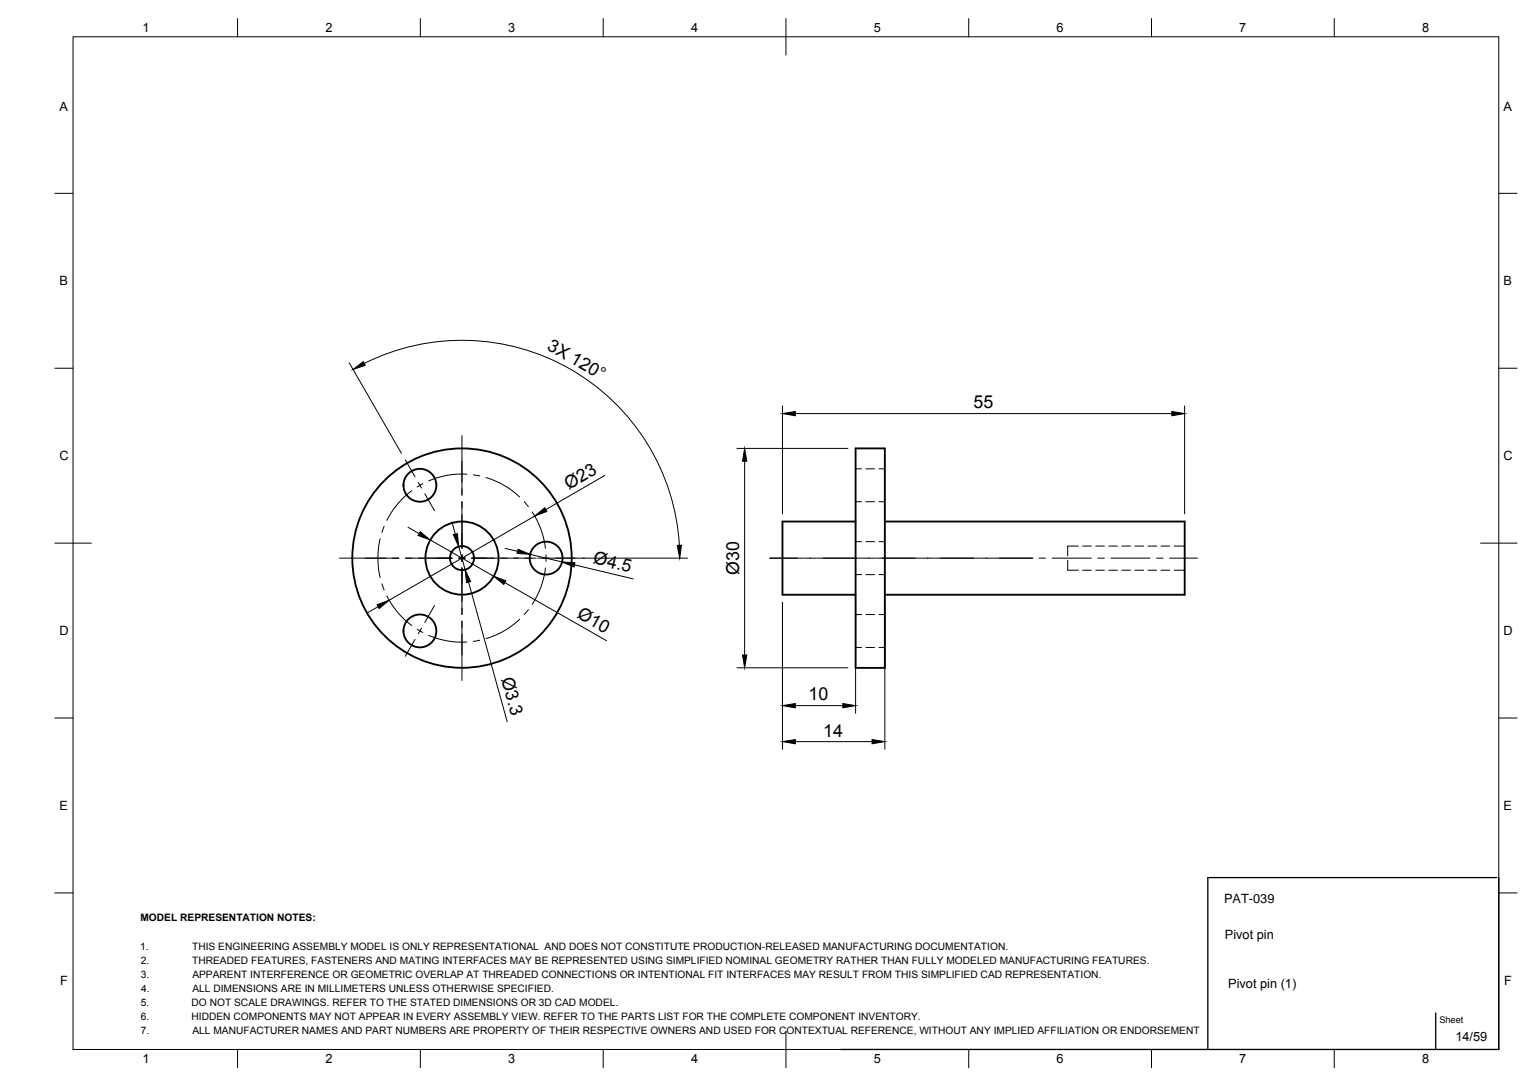
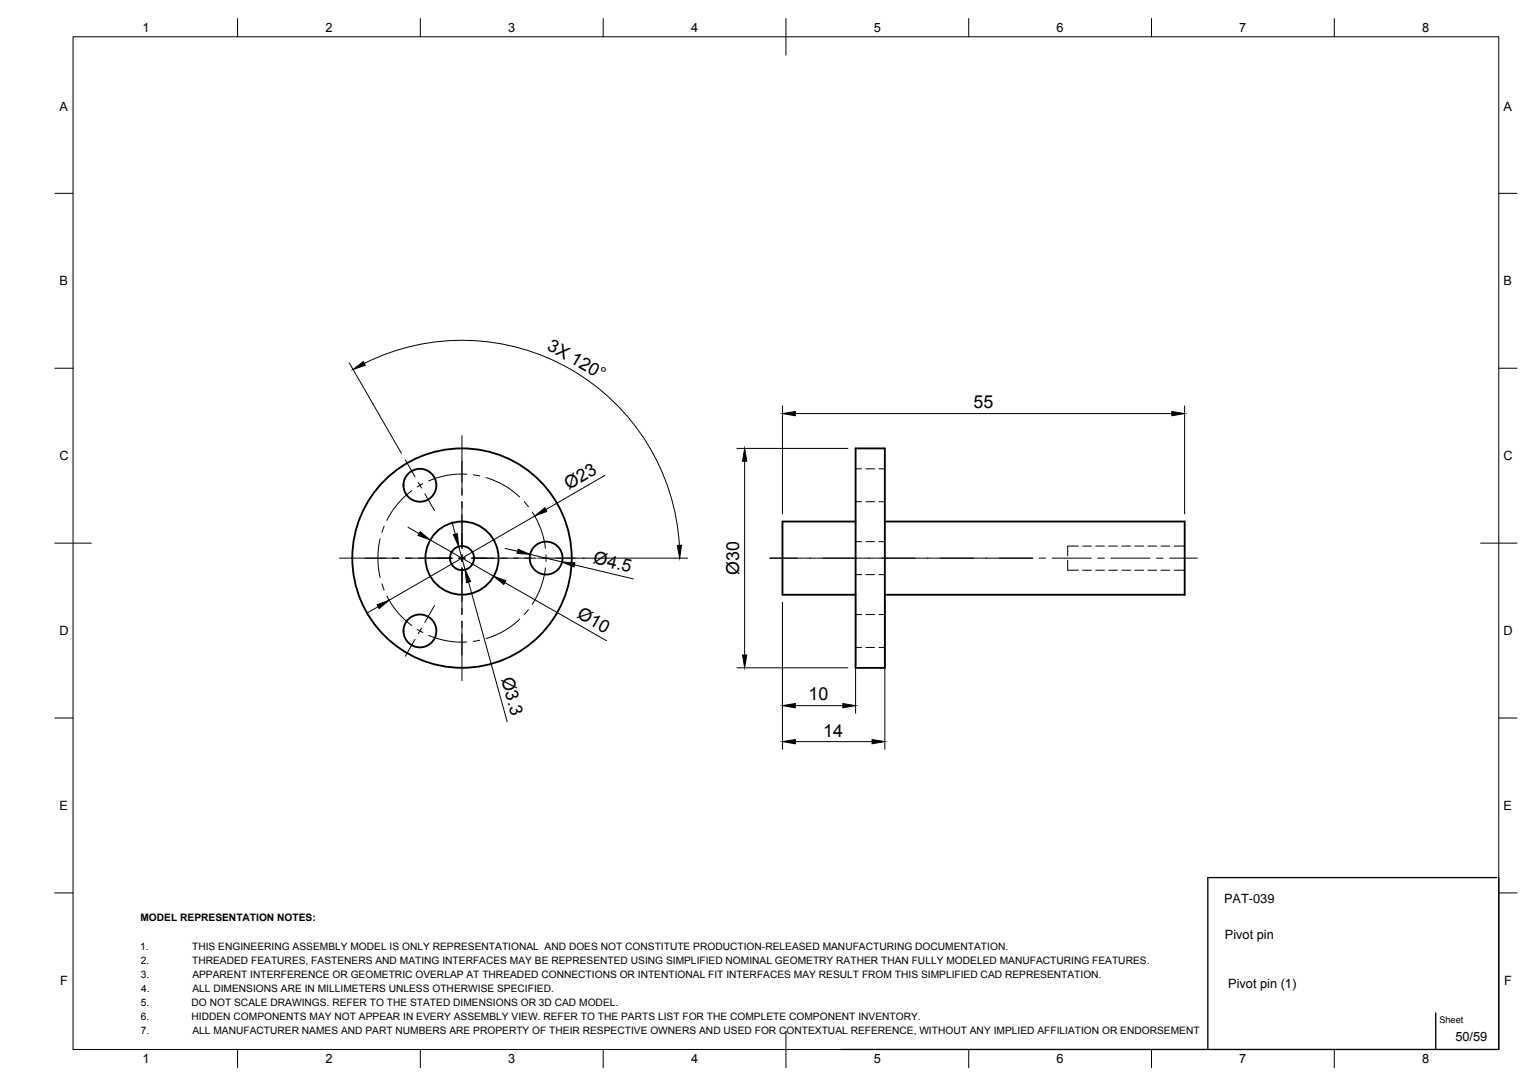
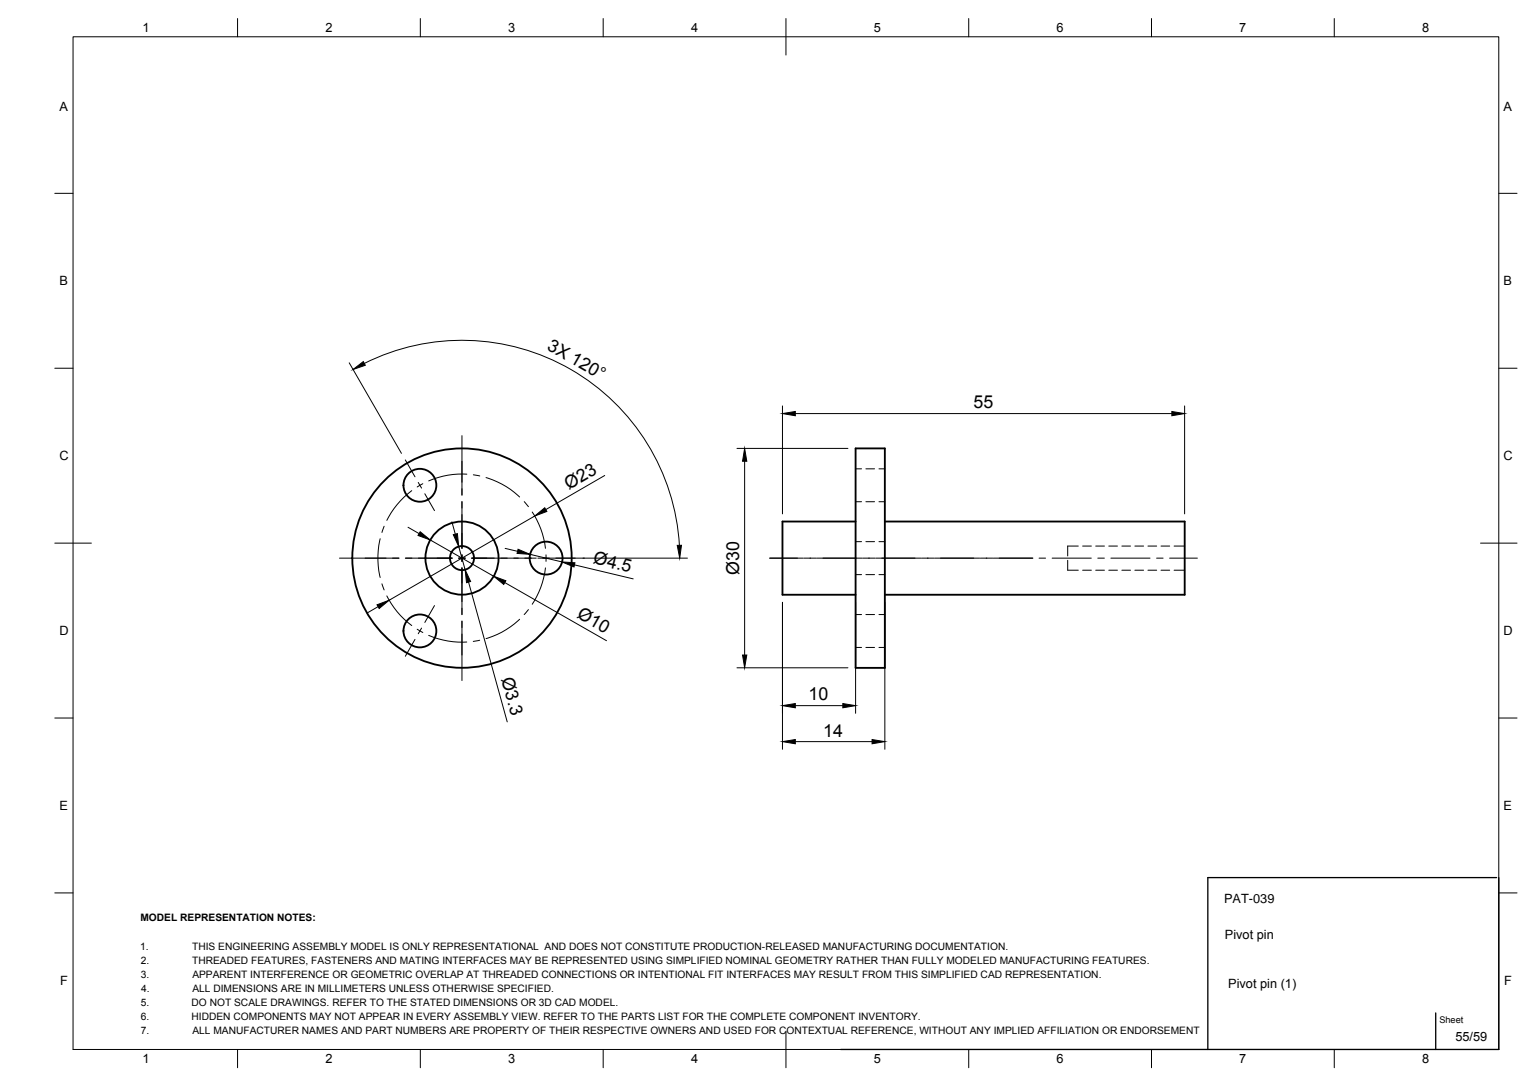
ISO-10303-21;
HEADER;
/* Generated by software containing ST-Developer
 * from STEP Tools, Inc. (www.steptools.com) 
 */

FILE_DESCRIPTION(
/* description */ ('Four-bar parallelogram arm'),
/* implementation_level */ '2;1');

FILE_NAME(
/* name */ 'Pivot pin.step',
/* time_stamp */ '2026-10-28T03:24:55-07:00',
/* author */ (''),
/* organization */ (''),
/* preprocessor_version */ 'ST-DEVELOPER v20.2',
/* originating_system */ 'Autodesk Translation Framework v15.17.0.0',
/* authorisation */ '');

FILE_SCHEMA (('AUTOMOTIVE_DESIGN { 1 0 10303 214 3 1 1 }'));
ENDSEC;

DATA;
#10=MECHANICAL_DESIGN_GEOMETRIC_PRESENTATION_REPRESENTATION('',(#631),#14512);
#531=SHAPE_REPRESENTATION_RELATIONSHIP('SRR','None',#14752,#581);
#581=ADVANCED_BREP_SHAPE_REPRESENTATION('',(#689),#14467);
#631=STYLED_ITEM('',(#15087),#689);
#689=MANIFOLD_SOLID_BREP('Body1',#7335);
#785=FACE_BOUND('',#1751,.T.);
#786=FACE_BOUND('',#1752,.T.);
#787=FACE_BOUND('',#1753,.T.);
#788=FACE_BOUND('',#1754,.T.);
#789=FACE_BOUND('',#1756,.T.);
#790=FACE_BOUND('',#1757,.T.);
#791=FACE_BOUND('',#1758,.T.);
#792=FACE_BOUND('',#1759,.T.);
#793=FACE_BOUND('',#1765,.T.);
#1048=PLANE('',#8091);
#1049=PLANE('',#8101);
#1050=PLANE('',#8104);
#1051=PLANE('',#8112);
#1052=PLANE('',#8113);
#1275=FACE_OUTER_BOUND('',#1745,.T.);
#1276=FACE_OUTER_BOUND('',#1746,.T.);
#1277=FACE_OUTER_BOUND('',#1747,.T.);
#1278=FACE_OUTER_BOUND('',#1748,.T.);
#1279=FACE_OUTER_BOUND('',#1749,.T.);
#1280=FACE_OUTER_BOUND('',#1750,.T.);
#1281=FACE_OUTER_BOUND('',#1755,.T.);
#1282=FACE_OUTER_BOUND('',#1760,.T.);
#1283=FACE_OUTER_BOUND('',#1761,.T.);
#1284=FACE_OUTER_BOUND('',#1762,.T.);
#1285=FACE_OUTER_BOUND('',#1763,.T.);
#1286=FACE_OUTER_BOUND('',#1764,.T.);
#1745=EDGE_LOOP('',(#5300,#5301,#5302,#5303));
#1746=EDGE_LOOP('',(#5304));
#1747=EDGE_LOOP('',(#5305,#5306,#5307,#5308));
#1748=EDGE_LOOP('',(#5309,#5310,#5311,#5312));
#1749=EDGE_LOOP('',(#5313,#5314,#5315,#5316));
#1750=EDGE_LOOP('',(#5317));
#1751=EDGE_LOOP('',(#5318));
#1752=EDGE_LOOP('',(#5319));
#1753=EDGE_LOOP('',(#5320));
#1754=EDGE_LOOP('',(#5321));
#1755=EDGE_LOOP('',(#5322));
#1756=EDGE_LOOP('',(#5323));
#1757=EDGE_LOOP('',(#5324));
#1758=EDGE_LOOP('',(#5325));
#1759=EDGE_LOOP('',(#5326));
#1760=EDGE_LOOP('',(#5327,#5328,#5329,#5330));
#1761=EDGE_LOOP('',(#5331,#5332,#5333,#5334));
#1762=EDGE_LOOP('',(#5335,#5336,#5337,#5338));
#1763=EDGE_LOOP('',(#5339));
#1764=EDGE_LOOP('',(#5340));
#1765=EDGE_LOOP('',(#5341));
#2404=LINE('',#11778,#2798);
#2405=LINE('',#11785,#2799);
#2406=LINE('',#11791,#2800);
#2407=LINE('',#11797,#2801);
#2408=LINE('',#11810,#2802);
#2409=LINE('',#11813,#2803);
#2410=LINE('',#11818,#2804);
#2798=VECTOR('',#9366,0.165);
#2799=VECTOR('',#9375,0.225);
#2800=VECTOR('',#9382,0.225);
#2801=VECTOR('',#9389,0.225);
#2802=VECTOR('',#9406,1.5);
#2803=VECTOR('',#9409,0.5);
#2804=VECTOR('',#9416,0.5);
#3164=CIRCLE('',#8089,0.165);
#3165=CIRCLE('',#8090,0.165);
#3166=CIRCLE('',#8093,0.225);
#3167=CIRCLE('',#8094,0.225);
#3168=CIRCLE('',#8096,0.225);
#3169=CIRCLE('',#8097,0.225);
#3170=CIRCLE('',#8099,0.225);
#3171=CIRCLE('',#8100,0.225);
#3172=CIRCLE('',#8102,1.5);
#3173=CIRCLE('',#8103,0.5);
#3174=CIRCLE('',#8105,1.5);
#3175=CIRCLE('',#8106,0.5);
#3176=CIRCLE('',#8109,0.5);
#3177=CIRCLE('',#8111,0.5);
#3649=VERTEX_POINT('',#11775);
#3650=VERTEX_POINT('',#11777);
#3651=VERTEX_POINT('',#11782);
#3652=VERTEX_POINT('',#11784);
#3653=VERTEX_POINT('',#11788);
#3654=VERTEX_POINT('',#11790);
#3655=VERTEX_POINT('',#11794);
#3656=VERTEX_POINT('',#11796);
#3657=VERTEX_POINT('',#11800);
#3658=VERTEX_POINT('',#11802);
#3659=VERTEX_POINT('',#11805);
#3660=VERTEX_POINT('',#11807);
#3661=VERTEX_POINT('',#11812);
#3662=VERTEX_POINT('',#11816);
#4281=EDGE_CURVE('',#3649,#3649,#3164,.T.);
#4282=EDGE_CURVE('',#3649,#3650,#2404,.T.);
#4283=EDGE_CURVE('',#3650,#3650,#3165,.T.);
#4284=EDGE_CURVE('',#3651,#3651,#3166,.T.);
#4285=EDGE_CURVE('',#3651,#3652,#2405,.T.);
#4286=EDGE_CURVE('',#3652,#3652,#3167,.T.);
#4287=EDGE_CURVE('',#3653,#3653,#3168,.T.);
#4288=EDGE_CURVE('',#3653,#3654,#2406,.T.);
#4289=EDGE_CURVE('',#3654,#3654,#3169,.T.);
#4290=EDGE_CURVE('',#3655,#3655,#3170,.T.);
#4291=EDGE_CURVE('',#3655,#3656,#2407,.T.);
#4292=EDGE_CURVE('',#3656,#3656,#3171,.T.);
#4293=EDGE_CURVE('',#3657,#3657,#3172,.T.);
#4294=EDGE_CURVE('',#3658,#3658,#3173,.T.);
#4295=EDGE_CURVE('',#3659,#3659,#3174,.T.);
#4296=EDGE_CURVE('',#3660,#3660,#3175,.T.);
#4297=EDGE_CURVE('',#3657,#3659,#2408,.T.);
#4298=EDGE_CURVE('',#3660,#3661,#2409,.T.);
#4299=EDGE_CURVE('',#3661,#3661,#3176,.T.);
#4300=EDGE_CURVE('',#3662,#3662,#3177,.T.);
#4301=EDGE_CURVE('',#3662,#3658,#2410,.T.);
#5300=ORIENTED_EDGE('',*,*,#4281,.F.);
#5301=ORIENTED_EDGE('',*,*,#4282,.T.);
#5302=ORIENTED_EDGE('',*,*,#4283,.T.);
#5303=ORIENTED_EDGE('',*,*,#4282,.F.);
#5304=ORIENTED_EDGE('',*,*,#4283,.F.);
#5305=ORIENTED_EDGE('',*,*,#4284,.F.);
#5306=ORIENTED_EDGE('',*,*,#4285,.T.);
#5307=ORIENTED_EDGE('',*,*,#4286,.F.);
#5308=ORIENTED_EDGE('',*,*,#4285,.F.);
#5309=ORIENTED_EDGE('',*,*,#4287,.F.);
#5310=ORIENTED_EDGE('',*,*,#4288,.T.);
#5311=ORIENTED_EDGE('',*,*,#4289,.F.);
#5312=ORIENTED_EDGE('',*,*,#4288,.F.);
#5313=ORIENTED_EDGE('',*,*,#4290,.F.);
#5314=ORIENTED_EDGE('',*,*,#4291,.T.);
#5315=ORIENTED_EDGE('',*,*,#4292,.F.);
#5316=ORIENTED_EDGE('',*,*,#4291,.F.);
#5317=ORIENTED_EDGE('',*,*,#4293,.T.);
#5318=ORIENTED_EDGE('',*,*,#4286,.T.);
#5319=ORIENTED_EDGE('',*,*,#4289,.T.);
#5320=ORIENTED_EDGE('',*,*,#4292,.T.);
#5321=ORIENTED_EDGE('',*,*,#4294,.F.);
#5322=ORIENTED_EDGE('',*,*,#4295,.F.);
#5323=ORIENTED_EDGE('',*,*,#4284,.T.);
#5324=ORIENTED_EDGE('',*,*,#4287,.T.);
#5325=ORIENTED_EDGE('',*,*,#4290,.T.);
#5326=ORIENTED_EDGE('',*,*,#4296,.F.);
#5327=ORIENTED_EDGE('',*,*,#4293,.F.);
#5328=ORIENTED_EDGE('',*,*,#4297,.T.);
#5329=ORIENTED_EDGE('',*,*,#4295,.T.);
#5330=ORIENTED_EDGE('',*,*,#4297,.F.);
#5331=ORIENTED_EDGE('',*,*,#4296,.T.);
#5332=ORIENTED_EDGE('',*,*,#4298,.T.);
#5333=ORIENTED_EDGE('',*,*,#4299,.T.);
#5334=ORIENTED_EDGE('',*,*,#4298,.F.);
#5335=ORIENTED_EDGE('',*,*,#4300,.F.);
#5336=ORIENTED_EDGE('',*,*,#4301,.T.);
#5337=ORIENTED_EDGE('',*,*,#4294,.T.);
#5338=ORIENTED_EDGE('',*,*,#4301,.F.);
#5339=ORIENTED_EDGE('',*,*,#4300,.T.);
#5340=ORIENTED_EDGE('',*,*,#4299,.F.);
#5341=ORIENTED_EDGE('',*,*,#4281,.T.);
#6746=CYLINDRICAL_SURFACE('',#8088,0.165);
#6747=CYLINDRICAL_SURFACE('',#8092,0.225);
#6748=CYLINDRICAL_SURFACE('',#8095,0.225);
#6749=CYLINDRICAL_SURFACE('',#8098,0.225);
#6750=CYLINDRICAL_SURFACE('',#8107,1.5);
#6751=CYLINDRICAL_SURFACE('',#8108,0.5);
#6752=CYLINDRICAL_SURFACE('',#8110,0.5);
#6980=ADVANCED_FACE('',(#1275),#6746,.F.);
#6981=ADVANCED_FACE('',(#1276),#1048,.F.);
#6982=ADVANCED_FACE('',(#1277),#6747,.F.);
#6983=ADVANCED_FACE('',(#1278),#6748,.F.);
#6984=ADVANCED_FACE('',(#1279),#6749,.F.);
#6985=ADVANCED_FACE('',(#1280,#785,#786,#787,#788),#1049,.T.);
#6986=ADVANCED_FACE('',(#1281,#789,#790,#791,#792),#1050,.F.);
#6987=ADVANCED_FACE('',(#1282),#6750,.T.);
#6988=ADVANCED_FACE('',(#1283),#6751,.T.);
#6989=ADVANCED_FACE('',(#1284),#6752,.T.);
#6990=ADVANCED_FACE('',(#1285),#1051,.T.);
#6991=ADVANCED_FACE('',(#1286,#793),#1052,.F.);
#7335=CLOSED_SHELL('',(#6980,#6981,#6982,#6983,#6984,#6985,#6986,#6987,
#6988,#6989,#6990,#6991));
#8087=AXIS2_PLACEMENT_3D('',#11773,#9360,#9361);
#8088=AXIS2_PLACEMENT_3D('',#11774,#9362,#9363);
#8089=AXIS2_PLACEMENT_3D('',#11776,#9364,#9365);
#8090=AXIS2_PLACEMENT_3D('',#11779,#9367,#9368);
#8091=AXIS2_PLACEMENT_3D('',#11780,#9369,#9370);
#8092=AXIS2_PLACEMENT_3D('',#11781,#9371,#9372);
#8093=AXIS2_PLACEMENT_3D('',#11783,#9373,#9374);
#8094=AXIS2_PLACEMENT_3D('',#11786,#9376,#9377);
#8095=AXIS2_PLACEMENT_3D('',#11787,#9378,#9379);
#8096=AXIS2_PLACEMENT_3D('',#11789,#9380,#9381);
#8097=AXIS2_PLACEMENT_3D('',#11792,#9383,#9384);
#8098=AXIS2_PLACEMENT_3D('',#11793,#9385,#9386);
#8099=AXIS2_PLACEMENT_3D('',#11795,#9387,#9388);
#8100=AXIS2_PLACEMENT_3D('',#11798,#9390,#9391);
#8101=AXIS2_PLACEMENT_3D('',#11799,#9392,#9393);
#8102=AXIS2_PLACEMENT_3D('',#11801,#9394,#9395);
#8103=AXIS2_PLACEMENT_3D('',#11803,#9396,#9397);
#8104=AXIS2_PLACEMENT_3D('',#11804,#9398,#9399);
#8105=AXIS2_PLACEMENT_3D('',#11806,#9400,#9401);
#8106=AXIS2_PLACEMENT_3D('',#11808,#9402,#9403);
#8107=AXIS2_PLACEMENT_3D('',#11809,#9404,#9405);
#8108=AXIS2_PLACEMENT_3D('',#11811,#9407,#9408);
#8109=AXIS2_PLACEMENT_3D('',#11814,#9410,#9411);
#8110=AXIS2_PLACEMENT_3D('',#11815,#9412,#9413);
#8111=AXIS2_PLACEMENT_3D('',#11817,#9414,#9415);
#8112=AXIS2_PLACEMENT_3D('',#11819,#9417,#9418);
#8113=AXIS2_PLACEMENT_3D('',#11820,#9419,#9420);
#9360=DIRECTION('axis',(0.,0.,1.));
#9361=DIRECTION('refdir',(1.,0.,0.));
#9362=DIRECTION('center_axis',(0.,1.,0.));
#9363=DIRECTION('ref_axis',(1.,0.,0.));
#9364=DIRECTION('center_axis',(0.,1.,0.));
#9365=DIRECTION('ref_axis',(1.,0.,0.));
#9366=DIRECTION('',(0.,1.,0.));
#9367=DIRECTION('center_axis',(0.,1.,0.));
#9368=DIRECTION('ref_axis',(1.,0.,0.));
#9369=DIRECTION('center_axis',(0.,1.,0.));
#9370=DIRECTION('ref_axis',(1.,0.,0.));
#9371=DIRECTION('center_axis',(0.,1.,0.));
#9372=DIRECTION('ref_axis',(1.,0.,0.));
#9373=DIRECTION('center_axis',(0.,1.,0.));
#9374=DIRECTION('ref_axis',(1.,0.,0.));
#9375=DIRECTION('',(0.,1.,0.));
#9376=DIRECTION('center_axis',(0.,-1.,0.));
#9377=DIRECTION('ref_axis',(1.,0.,0.));
#9378=DIRECTION('center_axis',(0.,1.,0.));
#9379=DIRECTION('ref_axis',(1.,0.,0.));
#9380=DIRECTION('center_axis',(0.,1.,0.));
#9381=DIRECTION('ref_axis',(1.,0.,0.));
#9382=DIRECTION('',(0.,1.,0.));
#9383=DIRECTION('center_axis',(0.,-1.,0.));
#9384=DIRECTION('ref_axis',(1.,0.,0.));
#9385=DIRECTION('center_axis',(0.,1.,0.));
#9386=DIRECTION('ref_axis',(1.,0.,0.));
#9387=DIRECTION('center_axis',(0.,1.,0.));
#9388=DIRECTION('ref_axis',(1.,0.,0.));
#9389=DIRECTION('',(0.,1.,0.));
#9390=DIRECTION('center_axis',(0.,-1.,0.));
#9391=DIRECTION('ref_axis',(1.,0.,0.));
#9392=DIRECTION('center_axis',(0.,1.,0.));
#9393=DIRECTION('ref_axis',(1.,0.,0.));
#9394=DIRECTION('center_axis',(0.,1.,0.));
#9395=DIRECTION('ref_axis',(1.,0.,0.));
#9396=DIRECTION('center_axis',(0.,1.,0.));
#9397=DIRECTION('ref_axis',(1.,0.,0.));
#9398=DIRECTION('center_axis',(0.,1.,0.));
#9399=DIRECTION('ref_axis',(1.,0.,0.));
#9400=DIRECTION('center_axis',(0.,1.,0.));
#9401=DIRECTION('ref_axis',(1.,0.,0.));
#9402=DIRECTION('center_axis',(0.,-1.,0.));
#9403=DIRECTION('ref_axis',(1.,0.,0.));
#9404=DIRECTION('center_axis',(0.,1.,0.));
#9405=DIRECTION('ref_axis',(1.,0.,0.));
#9406=DIRECTION('',(0.,-1.,0.));
#9407=DIRECTION('center_axis',(0.,1.,0.));
#9408=DIRECTION('ref_axis',(1.,0.,0.));
#9409=DIRECTION('',(0.,-1.,0.));
#9410=DIRECTION('center_axis',(0.,1.,0.));
#9411=DIRECTION('ref_axis',(1.,0.,0.));
#9412=DIRECTION('center_axis',(0.,1.,0.));
#9413=DIRECTION('ref_axis',(1.,0.,0.));
#9414=DIRECTION('center_axis',(0.,1.,0.));
#9415=DIRECTION('ref_axis',(1.,0.,0.));
#9416=DIRECTION('',(0.,-1.,0.));
#9417=DIRECTION('center_axis',(0.,1.,0.));
#9418=DIRECTION('ref_axis',(1.,0.,0.));
#9419=DIRECTION('center_axis',(0.,1.,0.));
#9420=DIRECTION('ref_axis',(1.,0.,0.));
#11773=CARTESIAN_POINT('',(0.,0.,0.));
#11774=CARTESIAN_POINT('Origin',(0.,-1.7,14.));
#11775=CARTESIAN_POINT('',(-0.165,-1.6,14.));
#11776=CARTESIAN_POINT('Origin',(0.,-1.6,14.));
#11777=CARTESIAN_POINT('',(-0.165,0.,14.));
#11778=CARTESIAN_POINT('',(-0.165,-1.7,14.));
#11779=CARTESIAN_POINT('Origin',(0.,0.,14.));
#11780=CARTESIAN_POINT('Origin',(0.,0.,14.));
#11781=CARTESIAN_POINT('Origin',(1.15,2.4,14.));
#11782=CARTESIAN_POINT('',(0.925,2.5,14.));
#11783=CARTESIAN_POINT('Origin',(1.15,2.5,14.));
#11784=CARTESIAN_POINT('',(0.925,2.9,14.));
#11785=CARTESIAN_POINT('',(0.925,2.4,14.));
#11786=CARTESIAN_POINT('Origin',(1.15,2.9,14.));
#11787=CARTESIAN_POINT('Origin',(-0.575,2.4,14.9959292143521));
#11788=CARTESIAN_POINT('',(-0.8,2.5,14.9959292143521));
#11789=CARTESIAN_POINT('Origin',(-0.575,2.5,14.9959292143521));
#11790=CARTESIAN_POINT('',(-0.8,2.9,14.9959292143521));
#11791=CARTESIAN_POINT('',(-0.8,2.4,14.9959292143521));
#11792=CARTESIAN_POINT('Origin',(-0.575,2.9,14.9959292143521));
#11793=CARTESIAN_POINT('Origin',(-0.575000000000001,2.4,13.0040707856479));
#11794=CARTESIAN_POINT('',(-0.8,2.5,13.0040707856479));
#11795=CARTESIAN_POINT('Origin',(-0.575000000000001,2.5,13.0040707856479));
#11796=CARTESIAN_POINT('',(-0.8,2.9,13.0040707856479));
#11797=CARTESIAN_POINT('',(-0.8,2.4,13.0040707856479));
#11798=CARTESIAN_POINT('Origin',(-0.575000000000001,2.9,13.0040707856479));
#11799=CARTESIAN_POINT('Origin',(0.,2.9,14.));
#11800=CARTESIAN_POINT('',(-1.5,2.9,14.));
#11801=CARTESIAN_POINT('Origin',(0.,2.9,14.));
#11802=CARTESIAN_POINT('',(-0.5,2.9,14.));
#11803=CARTESIAN_POINT('Origin',(0.,2.9,14.));
#11804=CARTESIAN_POINT('Origin',(0.,2.5,14.));
#11805=CARTESIAN_POINT('',(-1.5,2.5,14.));
#11806=CARTESIAN_POINT('Origin',(0.,2.5,14.));
#11807=CARTESIAN_POINT('',(-0.5,2.5,14.));
#11808=CARTESIAN_POINT('Origin',(0.,2.5,14.));
#11809=CARTESIAN_POINT('Origin',(0.,2.5,14.));
#11810=CARTESIAN_POINT('',(-1.5,2.5,14.));
#11811=CARTESIAN_POINT('Origin',(0.,-1.6,14.));
#11812=CARTESIAN_POINT('',(-0.5,-1.6,14.));
#11813=CARTESIAN_POINT('',(-0.5,-1.6,14.));
#11814=CARTESIAN_POINT('Origin',(0.,-1.6,14.));
#11815=CARTESIAN_POINT('Origin',(0.,-1.6,14.));
#11816=CARTESIAN_POINT('',(-0.5,3.9,14.));
#11817=CARTESIAN_POINT('Origin',(0.,3.9,14.));
#11818=CARTESIAN_POINT('',(-0.5,-1.6,14.));
#11819=CARTESIAN_POINT('Origin',(0.,3.9,14.));
#11820=CARTESIAN_POINT('Origin',(0.,-1.6,14.));
#14410=UNCERTAINTY_MEASURE_WITH_UNIT(LENGTH_MEASURE(0.001),#14513,
'DISTANCE_ACCURACY_VALUE',
'Maximum model space distance between geometric entities at asserted c
onnectivities');
#14455=UNCERTAINTY_MEASURE_WITH_UNIT(LENGTH_MEASURE(0.001),#14513,
'DISTANCE_ACCURACY_VALUE',
'Maximum model space distance between geometric entities at asserted c
onnectivities');
#14467=(
GEOMETRIC_REPRESENTATION_CONTEXT(3)
GLOBAL_UNCERTAINTY_ASSIGNED_CONTEXT((#14410))
GLOBAL_UNIT_ASSIGNED_CONTEXT((#14513,#14515,#14516))
REPRESENTATION_CONTEXT('','3D')
);
#14512=(
GEOMETRIC_REPRESENTATION_CONTEXT(3)
GLOBAL_UNCERTAINTY_ASSIGNED_CONTEXT((#14455))
GLOBAL_UNIT_ASSIGNED_CONTEXT((#14513,#14515,#14516))
REPRESENTATION_CONTEXT('','3D')
);
#14513=(
LENGTH_UNIT()
NAMED_UNIT(*)
SI_UNIT(.CENTI.,.METRE.)
);
#14515=(
NAMED_UNIT(*)
PLANE_ANGLE_UNIT()
SI_UNIT($,.RADIAN.)
);
#14516=(
NAMED_UNIT(*)
SI_UNIT($,.STERADIAN.)
SOLID_ANGLE_UNIT()
);
#14528=SHAPE_DEFINITION_REPRESENTATION(#14584,#14752);
#14584=PRODUCT_DEFINITION_SHAPE('',$,#14809);
#14752=SHAPE_REPRESENTATION('',(#8087),#14467);
#14797=PRODUCT_DEFINITION_CONTEXT('part definition',#14967,'design');
#14809=PRODUCT_DEFINITION('Pivot pin','Pivot pin',#14865,#14797);
#14865=PRODUCT_DEFINITION_FORMATION('',$,#14980);
#14967=APPLICATION_CONTEXT(
'Core Data for Automotive Mechanical Design Process');
#14968=PRODUCT_CONTEXT('part definition',#14967,'mechanical');
#14980=PRODUCT('Pivot pin','Pivot pin','Pivot pin',(#14968));
#15081=COLOUR_RGB('Grey',0.48,0.52,0.57);
#15082=FILL_AREA_STYLE_COLOUR('',#15081);
#15083=FILL_AREA_STYLE('',(#15082));
#15084=SURFACE_STYLE_FILL_AREA(#15083);
#15085=SURFACE_SIDE_STYLE('',(#15084));
#15086=SURFACE_STYLE_USAGE(.BOTH.,#15085);
#15087=PRESENTATION_STYLE_ASSIGNMENT((#15086));
ENDSEC;
END-ISO-10303-21;
